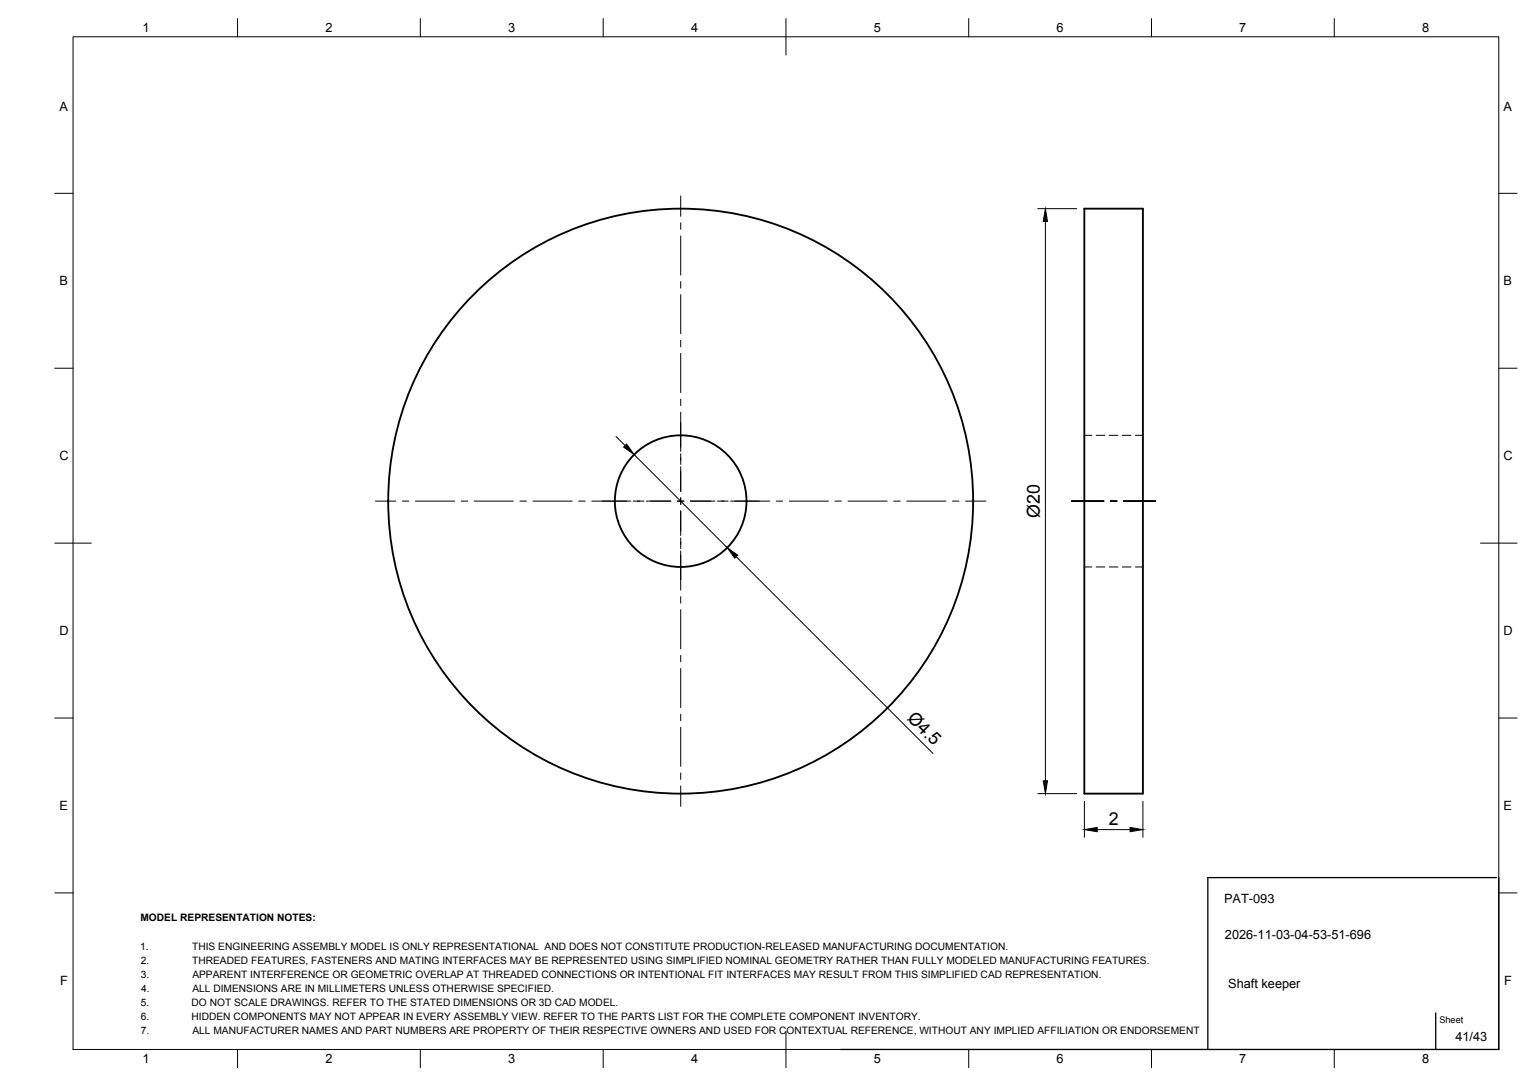
ISO-10303-21;
HEADER;
/* Generated by software containing ST-Developer
 * from STEP Tools, Inc. (www.steptools.com) 
 */

FILE_DESCRIPTION(
/* description */ ('Self-centering screw clamp'),
/* implementation_level */ '2;1');

FILE_NAME(
/* name */ 'Shaft keeper.step',
/* time_stamp */ '2026-10-28T03:25:31-07:00',
/* author */ (''),
/* organization */ (''),
/* preprocessor_version */ 'ST-DEVELOPER v20.2',
/* originating_system */ 'Autodesk Translation Framework v15.17.0.0',
/* authorisation */ '');

FILE_SCHEMA (('AUTOMOTIVE_DESIGN { 1 0 10303 214 3 1 1 }'));
ENDSEC;

DATA;
#10=MECHANICAL_DESIGN_GEOMETRIC_PRESENTATION_REPRESENTATION('',(#667),#16799);
#578=SHAPE_REPRESENTATION_RELATIONSHIP('SRR','None',#17056,#619);
#619=ADVANCED_BREP_SHAPE_REPRESENTATION('',(#714),#16794);
#667=STYLED_ITEM('',(#17326),#714);
#714=MANIFOLD_SOLID_BREP('Body1',#9119);
#1006=FACE_BOUND('',#2528,.T.);
#1007=FACE_BOUND('',#2530,.T.);
#1245=PLANE('',#10578);
#1246=PLANE('',#10579);
#1733=FACE_OUTER_BOUND('',#2525,.T.);
#1734=FACE_OUTER_BOUND('',#2526,.T.);
#1735=FACE_OUTER_BOUND('',#2527,.T.);
#1736=FACE_OUTER_BOUND('',#2529,.T.);
#2525=EDGE_LOOP('',(#8179,#8180,#8181,#8182));
#2526=EDGE_LOOP('',(#8183,#8184,#8185,#8186));
#2527=EDGE_LOOP('',(#8187));
#2528=EDGE_LOOP('',(#8188));
#2529=EDGE_LOOP('',(#8189));
#2530=EDGE_LOOP('',(#8190));
#3094=LINE('',#16343,#3667);
#3095=LINE('',#16349,#3668);
#3667=VECTOR('',#13263,0.225);
#3668=VECTOR('',#13270,1.);
#4207=CIRCLE('',#10573,0.225);
#4208=CIRCLE('',#10574,0.225);
#4209=CIRCLE('',#10576,1.);
#4210=CIRCLE('',#10577,1.);
#4919=VERTEX_POINT('',#16340);
#4920=VERTEX_POINT('',#16342);
#4921=VERTEX_POINT('',#16346);
#4922=VERTEX_POINT('',#16348);
#6014=EDGE_CURVE('',#4919,#4919,#4207,.T.);
#6015=EDGE_CURVE('',#4919,#4920,#3094,.T.);
#6016=EDGE_CURVE('',#4920,#4920,#4208,.T.);
#6017=EDGE_CURVE('',#4921,#4921,#4209,.T.);
#6018=EDGE_CURVE('',#4921,#4922,#3095,.T.);
#6019=EDGE_CURVE('',#4922,#4922,#4210,.T.);
#8179=ORIENTED_EDGE('',*,*,#6014,.F.);
#8180=ORIENTED_EDGE('',*,*,#6015,.T.);
#8181=ORIENTED_EDGE('',*,*,#6016,.T.);
#8182=ORIENTED_EDGE('',*,*,#6015,.F.);
#8183=ORIENTED_EDGE('',*,*,#6017,.F.);
#8184=ORIENTED_EDGE('',*,*,#6018,.T.);
#8185=ORIENTED_EDGE('',*,*,#6019,.T.);
#8186=ORIENTED_EDGE('',*,*,#6018,.F.);
#8187=ORIENTED_EDGE('',*,*,#6017,.T.);
#8188=ORIENTED_EDGE('',*,*,#6014,.T.);
#8189=ORIENTED_EDGE('',*,*,#6019,.F.);
#8190=ORIENTED_EDGE('',*,*,#6016,.F.);
#8561=CYLINDRICAL_SURFACE('',#10572,0.225);
#8562=CYLINDRICAL_SURFACE('',#10575,1.);
#9031=ADVANCED_FACE('',(#1733),#8561,.F.);
#9032=ADVANCED_FACE('',(#1734),#8562,.T.);
#9033=ADVANCED_FACE('',(#1735,#1006),#1245,.T.);
#9034=ADVANCED_FACE('',(#1736,#1007),#1246,.F.);
#9119=CLOSED_SHELL('',(#9031,#9032,#9033,#9034));
#10571=AXIS2_PLACEMENT_3D('',#16338,#13257,#13258);
#10572=AXIS2_PLACEMENT_3D('',#16339,#13259,#13260);
#10573=AXIS2_PLACEMENT_3D('',#16341,#13261,#13262);
#10574=AXIS2_PLACEMENT_3D('',#16344,#13264,#13265);
#10575=AXIS2_PLACEMENT_3D('',#16345,#13266,#13267);
#10576=AXIS2_PLACEMENT_3D('',#16347,#13268,#13269);
#10577=AXIS2_PLACEMENT_3D('',#16350,#13271,#13272);
#10578=AXIS2_PLACEMENT_3D('',#16351,#13273,#13274);
#10579=AXIS2_PLACEMENT_3D('',#16352,#13275,#13276);
#13257=DIRECTION('axis',(0.,0.,1.));
#13258=DIRECTION('refdir',(1.,0.,0.));
#13259=DIRECTION('center_axis',(1.,0.,0.));
#13260=DIRECTION('ref_axis',(0.,0.,-1.));
#13261=DIRECTION('center_axis',(-1.,0.,0.));
#13262=DIRECTION('ref_axis',(0.,0.,-1.));
#13263=DIRECTION('',(-1.,0.,0.));
#13264=DIRECTION('center_axis',(-1.,0.,0.));
#13265=DIRECTION('ref_axis',(0.,0.,-1.));
#13266=DIRECTION('center_axis',(1.,0.,0.));
#13267=DIRECTION('ref_axis',(0.,0.,-1.));
#13268=DIRECTION('center_axis',(1.,0.,0.));
#13269=DIRECTION('ref_axis',(0.,0.,-1.));
#13270=DIRECTION('',(-1.,0.,0.));
#13271=DIRECTION('center_axis',(1.,0.,0.));
#13272=DIRECTION('ref_axis',(0.,0.,-1.));
#13273=DIRECTION('center_axis',(1.,0.,0.));
#13274=DIRECTION('ref_axis',(0.,0.,-1.));
#13275=DIRECTION('center_axis',(1.,0.,0.));
#13276=DIRECTION('ref_axis',(0.,0.,-1.));
#16338=CARTESIAN_POINT('',(0.,0.,0.));
#16339=CARTESIAN_POINT('Origin',(-15.2,0.,4.));
#16340=CARTESIAN_POINT('',(-15.,-2.75545529808155E-17,4.225));
#16341=CARTESIAN_POINT('Origin',(-15.,0.,4.));
#16342=CARTESIAN_POINT('',(-15.2,-2.75545529808155E-17,4.225));
#16343=CARTESIAN_POINT('',(-15.2,-2.75545529808155E-17,4.225));
#16344=CARTESIAN_POINT('Origin',(-15.2,0.,4.));
#16345=CARTESIAN_POINT('Origin',(-15.2,0.,4.));
#16346=CARTESIAN_POINT('',(-15.,-1.22464679914735E-16,5.));
#16347=CARTESIAN_POINT('Origin',(-15.,0.,4.));
#16348=CARTESIAN_POINT('',(-15.2,-1.22464679914735E-16,5.));
#16349=CARTESIAN_POINT('',(-15.2,-1.22464679914735E-16,5.));
#16350=CARTESIAN_POINT('Origin',(-15.2,0.,4.));
#16351=CARTESIAN_POINT('Origin',(-15.,0.,4.));
#16352=CARTESIAN_POINT('Origin',(-15.2,0.,4.));
#16745=UNCERTAINTY_MEASURE_WITH_UNIT(LENGTH_MEASURE(0.001),#16800,
'DISTANCE_ACCURACY_VALUE',
'Maximum model space distance between geometric entities at asserted c
onnectivities');
#16750=UNCERTAINTY_MEASURE_WITH_UNIT(LENGTH_MEASURE(0.001),#16800,
'DISTANCE_ACCURACY_VALUE',
'Maximum model space distance between geometric entities at asserted c
onnectivities');
#16794=(
GEOMETRIC_REPRESENTATION_CONTEXT(3)
GLOBAL_UNCERTAINTY_ASSIGNED_CONTEXT((#16745))
GLOBAL_UNIT_ASSIGNED_CONTEXT((#16800,#16802,#16803))
REPRESENTATION_CONTEXT('','3D')
);
#16799=(
GEOMETRIC_REPRESENTATION_CONTEXT(3)
GLOBAL_UNCERTAINTY_ASSIGNED_CONTEXT((#16750))
GLOBAL_UNIT_ASSIGNED_CONTEXT((#16800,#16802,#16803))
REPRESENTATION_CONTEXT('','3D')
);
#16800=(
LENGTH_UNIT()
NAMED_UNIT(*)
SI_UNIT(.CENTI.,.METRE.)
);
#16802=(
NAMED_UNIT(*)
PLANE_ANGLE_UNIT()
SI_UNIT($,.RADIAN.)
);
#16803=(
NAMED_UNIT(*)
SI_UNIT($,.STERADIAN.)
SOLID_ANGLE_UNIT()
);
#16847=SHAPE_DEFINITION_REPRESENTATION(#16902,#17056);
#16902=PRODUCT_DEFINITION_SHAPE('',$,#17105);
#17056=SHAPE_REPRESENTATION('',(#10571),#16794);
#17061=PRODUCT_DEFINITION_CONTEXT('part definition',#17207,'design');
#17105=PRODUCT_DEFINITION('Shaft keeper','Shaft keeper',#17153,#17061);
#17153=PRODUCT_DEFINITION_FORMATION('',$,#17252);
#17207=APPLICATION_CONTEXT(
'Core Data for Automotive Mechanical Design Process');
#17208=PRODUCT_CONTEXT('part definition',#17207,'mechanical');
#17252=PRODUCT('Shaft keeper','Shaft keeper','Shaft keeper',(#17208));
#17320=COLOUR_RGB('Grey',0.48,0.52,0.57);
#17321=FILL_AREA_STYLE_COLOUR('',#17320);
#17322=FILL_AREA_STYLE('',(#17321));
#17323=SURFACE_STYLE_FILL_AREA(#17322);
#17324=SURFACE_SIDE_STYLE('',(#17323));
#17325=SURFACE_STYLE_USAGE(.BOTH.,#17324);
#17326=PRESENTATION_STYLE_ASSIGNMENT((#17325));
ENDSEC;
END-ISO-10303-21;
